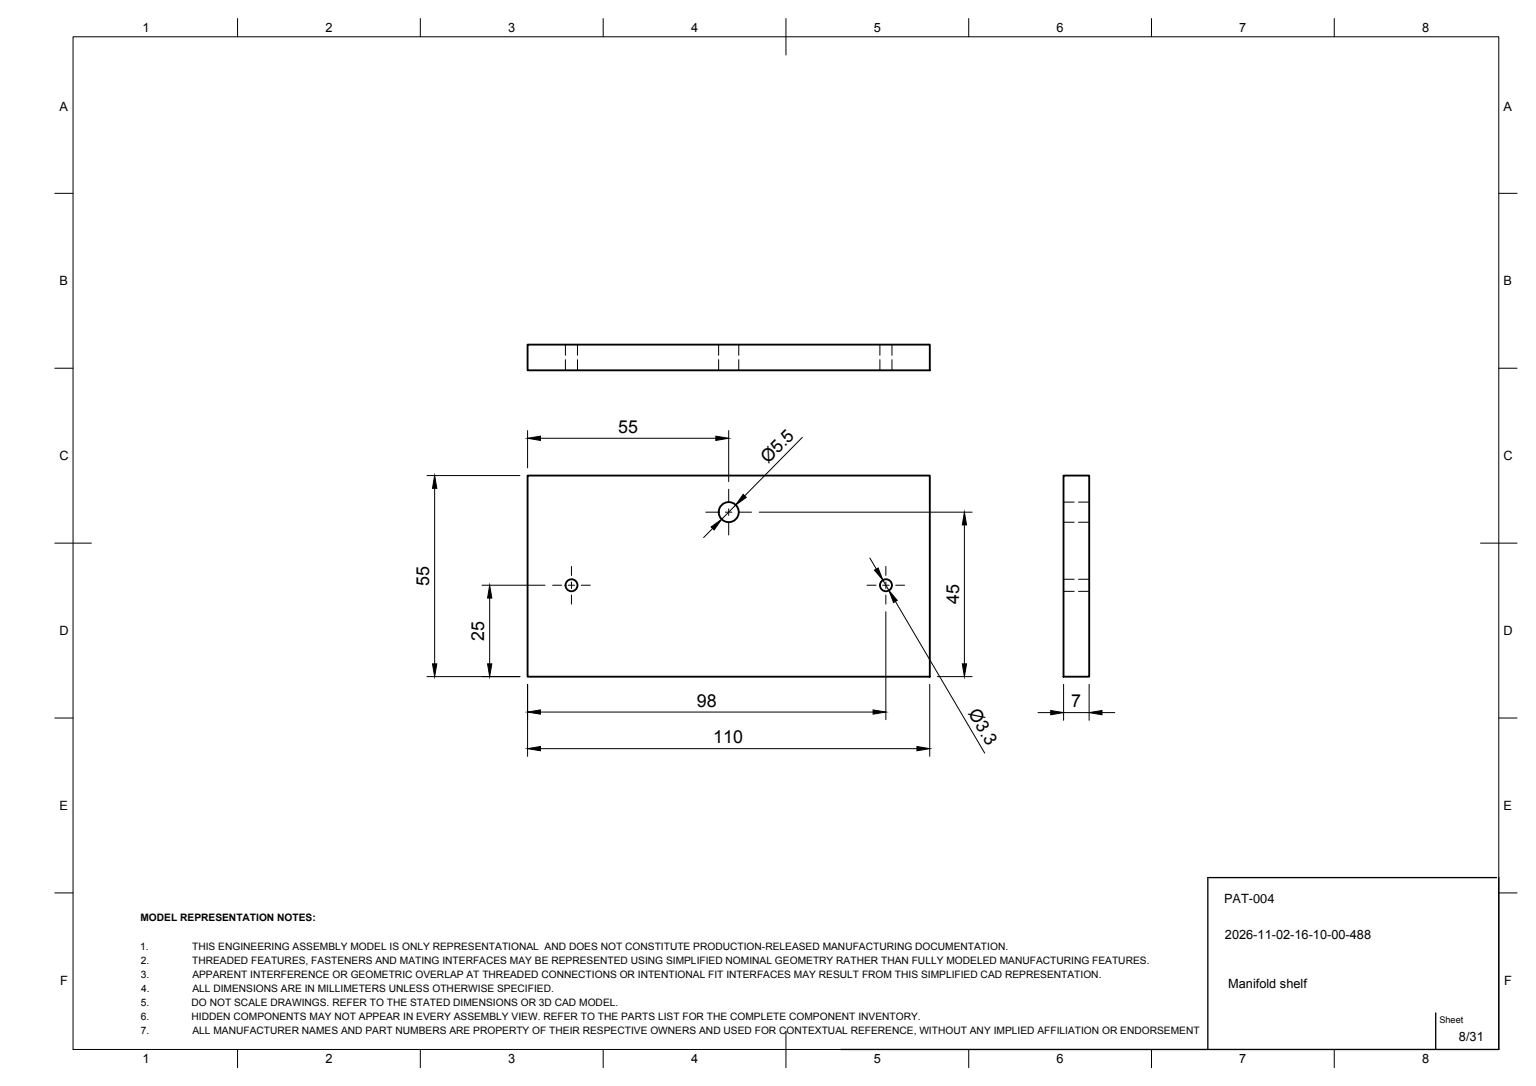
ISO-10303-21;
HEADER;
/* Generated by software containing ST-Developer
 * from STEP Tools, Inc. (www.steptools.com) 
 */

FILE_DESCRIPTION(
/* description */ ('Air blow-off nozzle station'),
/* implementation_level */ '2;1');

FILE_NAME(
/* name */ 'Manifold shelf.step',
/* time_stamp */ '2026-10-27T10:53:54-07:00',
/* author */ (''),
/* organization */ (''),
/* preprocessor_version */ 'ST-DEVELOPER v20.2',
/* originating_system */ 'Autodesk Translation Framework v15.17.0.0',
/* authorisation */ '');

FILE_SCHEMA (('AUTOMOTIVE_DESIGN { 1 0 10303 214 3 1 1 }'));
ENDSEC;

DATA;
#10=MECHANICAL_DESIGN_GEOMETRIC_PRESENTATION_REPRESENTATION('',(#240),#7897);
#190=SHAPE_REPRESENTATION_RELATIONSHIP('SRR','None',#8004,#215);
#215=ADVANCED_BREP_SHAPE_REPRESENTATION('',(#265),#7871);
#240=STYLED_ITEM('',(#8234),#265);
#265=MANIFOLD_SOLID_BREP('Body1',#4289);
#287=FACE_BOUND('',#825,.T.);
#288=FACE_BOUND('',#826,.T.);
#289=FACE_BOUND('',#827,.T.);
#290=FACE_BOUND('',#829,.T.);
#291=FACE_BOUND('',#830,.T.);
#292=FACE_BOUND('',#831,.T.);
#389=PLANE('',#4625);
#390=PLANE('',#4626);
#391=PLANE('',#4627);
#392=PLANE('',#4628);
#393=PLANE('',#4629);
#394=PLANE('',#4630);
#559=FACE_OUTER_BOUND('',#817,.T.);
#560=FACE_OUTER_BOUND('',#818,.T.);
#561=FACE_OUTER_BOUND('',#819,.T.);
#562=FACE_OUTER_BOUND('',#820,.T.);
#563=FACE_OUTER_BOUND('',#821,.T.);
#564=FACE_OUTER_BOUND('',#822,.T.);
#565=FACE_OUTER_BOUND('',#823,.T.);
#566=FACE_OUTER_BOUND('',#824,.T.);
#567=FACE_OUTER_BOUND('',#828,.T.);
#817=EDGE_LOOP('',(#2975,#2976,#2977,#2978));
#818=EDGE_LOOP('',(#2979,#2980,#2981,#2982));
#819=EDGE_LOOP('',(#2983,#2984,#2985,#2986));
#820=EDGE_LOOP('',(#2987,#2988,#2989,#2990));
#821=EDGE_LOOP('',(#2991,#2992,#2993,#2994));
#822=EDGE_LOOP('',(#2995,#2996,#2997,#2998));
#823=EDGE_LOOP('',(#2999,#3000,#3001,#3002));
#824=EDGE_LOOP('',(#3003,#3004,#3005,#3006));
#825=EDGE_LOOP('',(#3007));
#826=EDGE_LOOP('',(#3008));
#827=EDGE_LOOP('',(#3009));
#828=EDGE_LOOP('',(#3010,#3011,#3012,#3013));
#829=EDGE_LOOP('',(#3014));
#830=EDGE_LOOP('',(#3015));
#831=EDGE_LOOP('',(#3016));
#1175=LINE('',#6486,#1529);
#1176=LINE('',#6492,#1530);
#1177=LINE('',#6498,#1531);
#1178=LINE('',#6503,#1532);
#1179=LINE('',#6505,#1533);
#1180=LINE('',#6507,#1534);
#1181=LINE('',#6508,#1535);
#1182=LINE('',#6511,#1536);
#1183=LINE('',#6513,#1537);
#1184=LINE('',#6514,#1538);
#1185=LINE('',#6517,#1539);
#1186=LINE('',#6519,#1540);
#1187=LINE('',#6520,#1541);
#1188=LINE('',#6522,#1542);
#1189=LINE('',#6523,#1543);
#1529=VECTOR('',#5167,0.165);
#1530=VECTOR('',#5174,0.165);
#1531=VECTOR('',#5181,0.275);
#1532=VECTOR('',#5186,1.);
#1533=VECTOR('',#5187,1.);
#1534=VECTOR('',#5188,1.);
#1535=VECTOR('',#5189,1.);
#1536=VECTOR('',#5192,1.);
#1537=VECTOR('',#5193,1.);
#1538=VECTOR('',#5194,1.);
#1539=VECTOR('',#5197,1.);
#1540=VECTOR('',#5198,1.);
#1541=VECTOR('',#5199,1.);
#1542=VECTOR('',#5202,1.);
#1543=VECTOR('',#5203,1.);
#1848=CIRCLE('',#4617,0.165);
#1849=CIRCLE('',#4618,0.165);
#1850=CIRCLE('',#4620,0.165);
#1851=CIRCLE('',#4621,0.165);
#1852=CIRCLE('',#4623,0.275);
#1853=CIRCLE('',#4624,0.275);
#2033=VERTEX_POINT('',#6483);
#2034=VERTEX_POINT('',#6485);
#2035=VERTEX_POINT('',#6489);
#2036=VERTEX_POINT('',#6491);
#2037=VERTEX_POINT('',#6495);
#2038=VERTEX_POINT('',#6497);
#2039=VERTEX_POINT('',#6501);
#2040=VERTEX_POINT('',#6502);
#2041=VERTEX_POINT('',#6504);
#2042=VERTEX_POINT('',#6506);
#2043=VERTEX_POINT('',#6510);
#2044=VERTEX_POINT('',#6512);
#2045=VERTEX_POINT('',#6516);
#2046=VERTEX_POINT('',#6518);
#2405=EDGE_CURVE('',#2033,#2033,#1848,.T.);
#2406=EDGE_CURVE('',#2033,#2034,#1175,.T.);
#2407=EDGE_CURVE('',#2034,#2034,#1849,.T.);
#2408=EDGE_CURVE('',#2035,#2035,#1850,.T.);
#2409=EDGE_CURVE('',#2035,#2036,#1176,.T.);
#2410=EDGE_CURVE('',#2036,#2036,#1851,.T.);
#2411=EDGE_CURVE('',#2037,#2037,#1852,.T.);
#2412=EDGE_CURVE('',#2037,#2038,#1177,.T.);
#2413=EDGE_CURVE('',#2038,#2038,#1853,.T.);
#2414=EDGE_CURVE('',#2039,#2040,#1178,.T.);
#2415=EDGE_CURVE('',#2040,#2041,#1179,.T.);
#2416=EDGE_CURVE('',#2042,#2041,#1180,.T.);
#2417=EDGE_CURVE('',#2039,#2042,#1181,.T.);
#2418=EDGE_CURVE('',#2043,#2039,#1182,.T.);
#2419=EDGE_CURVE('',#2044,#2042,#1183,.T.);
#2420=EDGE_CURVE('',#2043,#2044,#1184,.T.);
#2421=EDGE_CURVE('',#2045,#2043,#1185,.T.);
#2422=EDGE_CURVE('',#2046,#2044,#1186,.T.);
#2423=EDGE_CURVE('',#2045,#2046,#1187,.T.);
#2424=EDGE_CURVE('',#2040,#2045,#1188,.T.);
#2425=EDGE_CURVE('',#2041,#2046,#1189,.T.);
#2975=ORIENTED_EDGE('',*,*,#2405,.F.);
#2976=ORIENTED_EDGE('',*,*,#2406,.T.);
#2977=ORIENTED_EDGE('',*,*,#2407,.F.);
#2978=ORIENTED_EDGE('',*,*,#2406,.F.);
#2979=ORIENTED_EDGE('',*,*,#2408,.F.);
#2980=ORIENTED_EDGE('',*,*,#2409,.T.);
#2981=ORIENTED_EDGE('',*,*,#2410,.F.);
#2982=ORIENTED_EDGE('',*,*,#2409,.F.);
#2983=ORIENTED_EDGE('',*,*,#2411,.F.);
#2984=ORIENTED_EDGE('',*,*,#2412,.T.);
#2985=ORIENTED_EDGE('',*,*,#2413,.F.);
#2986=ORIENTED_EDGE('',*,*,#2412,.F.);
#2987=ORIENTED_EDGE('',*,*,#2414,.T.);
#2988=ORIENTED_EDGE('',*,*,#2415,.T.);
#2989=ORIENTED_EDGE('',*,*,#2416,.F.);
#2990=ORIENTED_EDGE('',*,*,#2417,.F.);
#2991=ORIENTED_EDGE('',*,*,#2418,.T.);
#2992=ORIENTED_EDGE('',*,*,#2417,.T.);
#2993=ORIENTED_EDGE('',*,*,#2419,.F.);
#2994=ORIENTED_EDGE('',*,*,#2420,.F.);
#2995=ORIENTED_EDGE('',*,*,#2421,.T.);
#2996=ORIENTED_EDGE('',*,*,#2420,.T.);
#2997=ORIENTED_EDGE('',*,*,#2422,.F.);
#2998=ORIENTED_EDGE('',*,*,#2423,.F.);
#2999=ORIENTED_EDGE('',*,*,#2424,.T.);
#3000=ORIENTED_EDGE('',*,*,#2423,.T.);
#3001=ORIENTED_EDGE('',*,*,#2425,.F.);
#3002=ORIENTED_EDGE('',*,*,#2415,.F.);
#3003=ORIENTED_EDGE('',*,*,#2425,.T.);
#3004=ORIENTED_EDGE('',*,*,#2422,.T.);
#3005=ORIENTED_EDGE('',*,*,#2419,.T.);
#3006=ORIENTED_EDGE('',*,*,#2416,.T.);
#3007=ORIENTED_EDGE('',*,*,#2407,.T.);
#3008=ORIENTED_EDGE('',*,*,#2410,.T.);
#3009=ORIENTED_EDGE('',*,*,#2413,.T.);
#3010=ORIENTED_EDGE('',*,*,#2424,.F.);
#3011=ORIENTED_EDGE('',*,*,#2414,.F.);
#3012=ORIENTED_EDGE('',*,*,#2418,.F.);
#3013=ORIENTED_EDGE('',*,*,#2421,.F.);
#3014=ORIENTED_EDGE('',*,*,#2405,.T.);
#3015=ORIENTED_EDGE('',*,*,#2408,.T.);
#3016=ORIENTED_EDGE('',*,*,#2411,.T.);
#3960=CYLINDRICAL_SURFACE('',#4616,0.165);
#3961=CYLINDRICAL_SURFACE('',#4619,0.165);
#3962=CYLINDRICAL_SURFACE('',#4622,0.275);
#4049=ADVANCED_FACE('',(#559),#3960,.F.);
#4050=ADVANCED_FACE('',(#560),#3961,.F.);
#4051=ADVANCED_FACE('',(#561),#3962,.F.);
#4052=ADVANCED_FACE('',(#562),#389,.T.);
#4053=ADVANCED_FACE('',(#563),#390,.T.);
#4054=ADVANCED_FACE('',(#564),#391,.T.);
#4055=ADVANCED_FACE('',(#565),#392,.T.);
#4056=ADVANCED_FACE('',(#566,#287,#288,#289),#393,.T.);
#4057=ADVANCED_FACE('',(#567,#290,#291,#292),#394,.F.);
#4289=CLOSED_SHELL('',(#4049,#4050,#4051,#4052,#4053,#4054,#4055,#4056,
#4057));
#4615=AXIS2_PLACEMENT_3D('',#6481,#5161,#5162);
#4616=AXIS2_PLACEMENT_3D('',#6482,#5163,#5164);
#4617=AXIS2_PLACEMENT_3D('',#6484,#5165,#5166);
#4618=AXIS2_PLACEMENT_3D('',#6487,#5168,#5169);
#4619=AXIS2_PLACEMENT_3D('',#6488,#5170,#5171);
#4620=AXIS2_PLACEMENT_3D('',#6490,#5172,#5173);
#4621=AXIS2_PLACEMENT_3D('',#6493,#5175,#5176);
#4622=AXIS2_PLACEMENT_3D('',#6494,#5177,#5178);
#4623=AXIS2_PLACEMENT_3D('',#6496,#5179,#5180);
#4624=AXIS2_PLACEMENT_3D('',#6499,#5182,#5183);
#4625=AXIS2_PLACEMENT_3D('',#6500,#5184,#5185);
#4626=AXIS2_PLACEMENT_3D('',#6509,#5190,#5191);
#4627=AXIS2_PLACEMENT_3D('',#6515,#5195,#5196);
#4628=AXIS2_PLACEMENT_3D('',#6521,#5200,#5201);
#4629=AXIS2_PLACEMENT_3D('',#6524,#5204,#5205);
#4630=AXIS2_PLACEMENT_3D('',#6525,#5206,#5207);
#5161=DIRECTION('axis',(0.,0.,1.));
#5162=DIRECTION('refdir',(1.,0.,0.));
#5163=DIRECTION('center_axis',(0.,0.,1.));
#5164=DIRECTION('ref_axis',(1.,0.,0.));
#5165=DIRECTION('center_axis',(0.,0.,1.));
#5166=DIRECTION('ref_axis',(1.,0.,0.));
#5167=DIRECTION('',(0.,0.,1.));
#5168=DIRECTION('center_axis',(0.,0.,-1.));
#5169=DIRECTION('ref_axis',(1.,0.,0.));
#5170=DIRECTION('center_axis',(0.,0.,1.));
#5171=DIRECTION('ref_axis',(1.,0.,0.));
#5172=DIRECTION('center_axis',(0.,0.,1.));
#5173=DIRECTION('ref_axis',(1.,0.,0.));
#5174=DIRECTION('',(0.,0.,1.));
#5175=DIRECTION('center_axis',(0.,0.,-1.));
#5176=DIRECTION('ref_axis',(1.,0.,0.));
#5177=DIRECTION('center_axis',(0.,0.,1.));
#5178=DIRECTION('ref_axis',(1.,0.,0.));
#5179=DIRECTION('center_axis',(0.,0.,1.));
#5180=DIRECTION('ref_axis',(1.,0.,0.));
#5181=DIRECTION('',(0.,0.,1.));
#5182=DIRECTION('center_axis',(0.,0.,-1.));
#5183=DIRECTION('ref_axis',(1.,0.,0.));
#5184=DIRECTION('center_axis',(0.,1.,0.));
#5185=DIRECTION('ref_axis',(-1.,0.,0.));
#5186=DIRECTION('',(-1.,0.,0.));
#5187=DIRECTION('',(0.,0.,1.));
#5188=DIRECTION('',(-1.,0.,0.));
#5189=DIRECTION('',(0.,0.,1.));
#5190=DIRECTION('center_axis',(1.,0.,0.));
#5191=DIRECTION('ref_axis',(0.,1.,0.));
#5192=DIRECTION('',(0.,1.,0.));
#5193=DIRECTION('',(0.,1.,0.));
#5194=DIRECTION('',(0.,0.,1.));
#5195=DIRECTION('center_axis',(0.,-1.,0.));
#5196=DIRECTION('ref_axis',(1.,0.,0.));
#5197=DIRECTION('',(1.,0.,0.));
#5198=DIRECTION('',(1.,0.,0.));
#5199=DIRECTION('',(0.,0.,1.));
#5200=DIRECTION('center_axis',(-1.,0.,0.));
#5201=DIRECTION('ref_axis',(0.,-1.,0.));
#5202=DIRECTION('',(0.,-1.,0.));
#5203=DIRECTION('',(0.,-1.,0.));
#5204=DIRECTION('center_axis',(0.,0.,1.));
#5205=DIRECTION('ref_axis',(1.,0.,0.));
#5206=DIRECTION('center_axis',(0.,0.,1.));
#5207=DIRECTION('ref_axis',(1.,0.,0.));
#6481=CARTESIAN_POINT('',(0.,0.,0.));
#6482=CARTESIAN_POINT('Origin',(-4.3,1.,20.7));
#6483=CARTESIAN_POINT('',(-4.465,1.,20.8));
#6484=CARTESIAN_POINT('Origin',(-4.3,1.,20.8));
#6485=CARTESIAN_POINT('',(-4.465,1.,21.5));
#6486=CARTESIAN_POINT('',(-4.465,1.,20.7));
#6487=CARTESIAN_POINT('Origin',(-4.3,1.,21.5));
#6488=CARTESIAN_POINT('Origin',(4.3,1.,20.7));
#6489=CARTESIAN_POINT('',(4.135,1.,20.8));
#6490=CARTESIAN_POINT('Origin',(4.3,1.,20.8));
#6491=CARTESIAN_POINT('',(4.135,1.,21.5));
#6492=CARTESIAN_POINT('',(4.135,1.,20.7));
#6493=CARTESIAN_POINT('Origin',(4.3,1.,21.5));
#6494=CARTESIAN_POINT('Origin',(0.,3.,20.7));
#6495=CARTESIAN_POINT('',(-0.275,3.,20.8));
#6496=CARTESIAN_POINT('Origin',(0.,3.,20.8));
#6497=CARTESIAN_POINT('',(-0.275,3.,21.5));
#6498=CARTESIAN_POINT('',(-0.275,3.,20.7));
#6499=CARTESIAN_POINT('Origin',(0.,3.,21.5));
#6500=CARTESIAN_POINT('Origin',(5.5,4.,20.8));
#6501=CARTESIAN_POINT('',(5.5,4.,20.8));
#6502=CARTESIAN_POINT('',(-5.5,4.,20.8));
#6503=CARTESIAN_POINT('',(5.5,4.,20.8));
#6504=CARTESIAN_POINT('',(-5.5,4.,21.5));
#6505=CARTESIAN_POINT('',(-5.5,4.,20.8));
#6506=CARTESIAN_POINT('',(5.5,4.,21.5));
#6507=CARTESIAN_POINT('',(5.5,4.,21.5));
#6508=CARTESIAN_POINT('',(5.5,4.,20.8));
#6509=CARTESIAN_POINT('Origin',(5.5,-1.5,20.8));
#6510=CARTESIAN_POINT('',(5.5,-1.5,20.8));
#6511=CARTESIAN_POINT('',(5.5,-1.5,20.8));
#6512=CARTESIAN_POINT('',(5.5,-1.5,21.5));
#6513=CARTESIAN_POINT('',(5.5,-1.5,21.5));
#6514=CARTESIAN_POINT('',(5.5,-1.5,20.8));
#6515=CARTESIAN_POINT('Origin',(-5.5,-1.5,20.8));
#6516=CARTESIAN_POINT('',(-5.5,-1.5,20.8));
#6517=CARTESIAN_POINT('',(-5.5,-1.5,20.8));
#6518=CARTESIAN_POINT('',(-5.5,-1.5,21.5));
#6519=CARTESIAN_POINT('',(-5.5,-1.5,21.5));
#6520=CARTESIAN_POINT('',(-5.5,-1.5,20.8));
#6521=CARTESIAN_POINT('Origin',(-5.5,4.,20.8));
#6522=CARTESIAN_POINT('',(-5.5,4.,20.8));
#6523=CARTESIAN_POINT('',(-5.5,4.,21.5));
#6524=CARTESIAN_POINT('Origin',(0.,1.25,21.5));
#6525=CARTESIAN_POINT('Origin',(0.,1.25,20.8));
#7839=UNCERTAINTY_MEASURE_WITH_UNIT(LENGTH_MEASURE(0.001),#7898,
'DISTANCE_ACCURACY_VALUE',
'Maximum model space distance between geometric entities at asserted c
onnectivities');
#7865=UNCERTAINTY_MEASURE_WITH_UNIT(LENGTH_MEASURE(0.001),#7898,
'DISTANCE_ACCURACY_VALUE',
'Maximum model space distance between geometric entities at asserted c
onnectivities');
#7871=(
GEOMETRIC_REPRESENTATION_CONTEXT(3)
GLOBAL_UNCERTAINTY_ASSIGNED_CONTEXT((#7839))
GLOBAL_UNIT_ASSIGNED_CONTEXT((#7898,#7900,#7901))
REPRESENTATION_CONTEXT('','3D')
);
#7897=(
GEOMETRIC_REPRESENTATION_CONTEXT(3)
GLOBAL_UNCERTAINTY_ASSIGNED_CONTEXT((#7865))
GLOBAL_UNIT_ASSIGNED_CONTEXT((#7898,#7900,#7901))
REPRESENTATION_CONTEXT('','3D')
);
#7898=(
LENGTH_UNIT()
NAMED_UNIT(*)
SI_UNIT(.CENTI.,.METRE.)
);
#7900=(
NAMED_UNIT(*)
PLANE_ANGLE_UNIT()
SI_UNIT($,.RADIAN.)
);
#7901=(
NAMED_UNIT(*)
SI_UNIT($,.STERADIAN.)
SOLID_ANGLE_UNIT()
);
#7907=SHAPE_DEFINITION_REPRESENTATION(#7938,#8004);
#7938=PRODUCT_DEFINITION_SHAPE('',$,#8036);
#8004=SHAPE_REPRESENTATION('',(#4615),#7871);
#8030=PRODUCT_DEFINITION_CONTEXT('part definition',#8125,'design');
#8036=PRODUCT_DEFINITION('Manifold shelf','Manifold shelf',#8067,#8030);
#8067=PRODUCT_DEFINITION_FORMATION('',$,#8132);
#8125=APPLICATION_CONTEXT(
'Core Data for Automotive Mechanical Design Process');
#8126=PRODUCT_CONTEXT('part definition',#8125,'mechanical');
#8132=PRODUCT('Manifold shelf','Manifold shelf','Manifold shelf',(#8126));
#8228=COLOUR_RGB('Off White',0.89,0.88,0.83);
#8229=FILL_AREA_STYLE_COLOUR('',#8228);
#8230=FILL_AREA_STYLE('',(#8229));
#8231=SURFACE_STYLE_FILL_AREA(#8230);
#8232=SURFACE_SIDE_STYLE('',(#8231));
#8233=SURFACE_STYLE_USAGE(.BOTH.,#8232);
#8234=PRESENTATION_STYLE_ASSIGNMENT((#8233));
ENDSEC;
END-ISO-10303-21;
